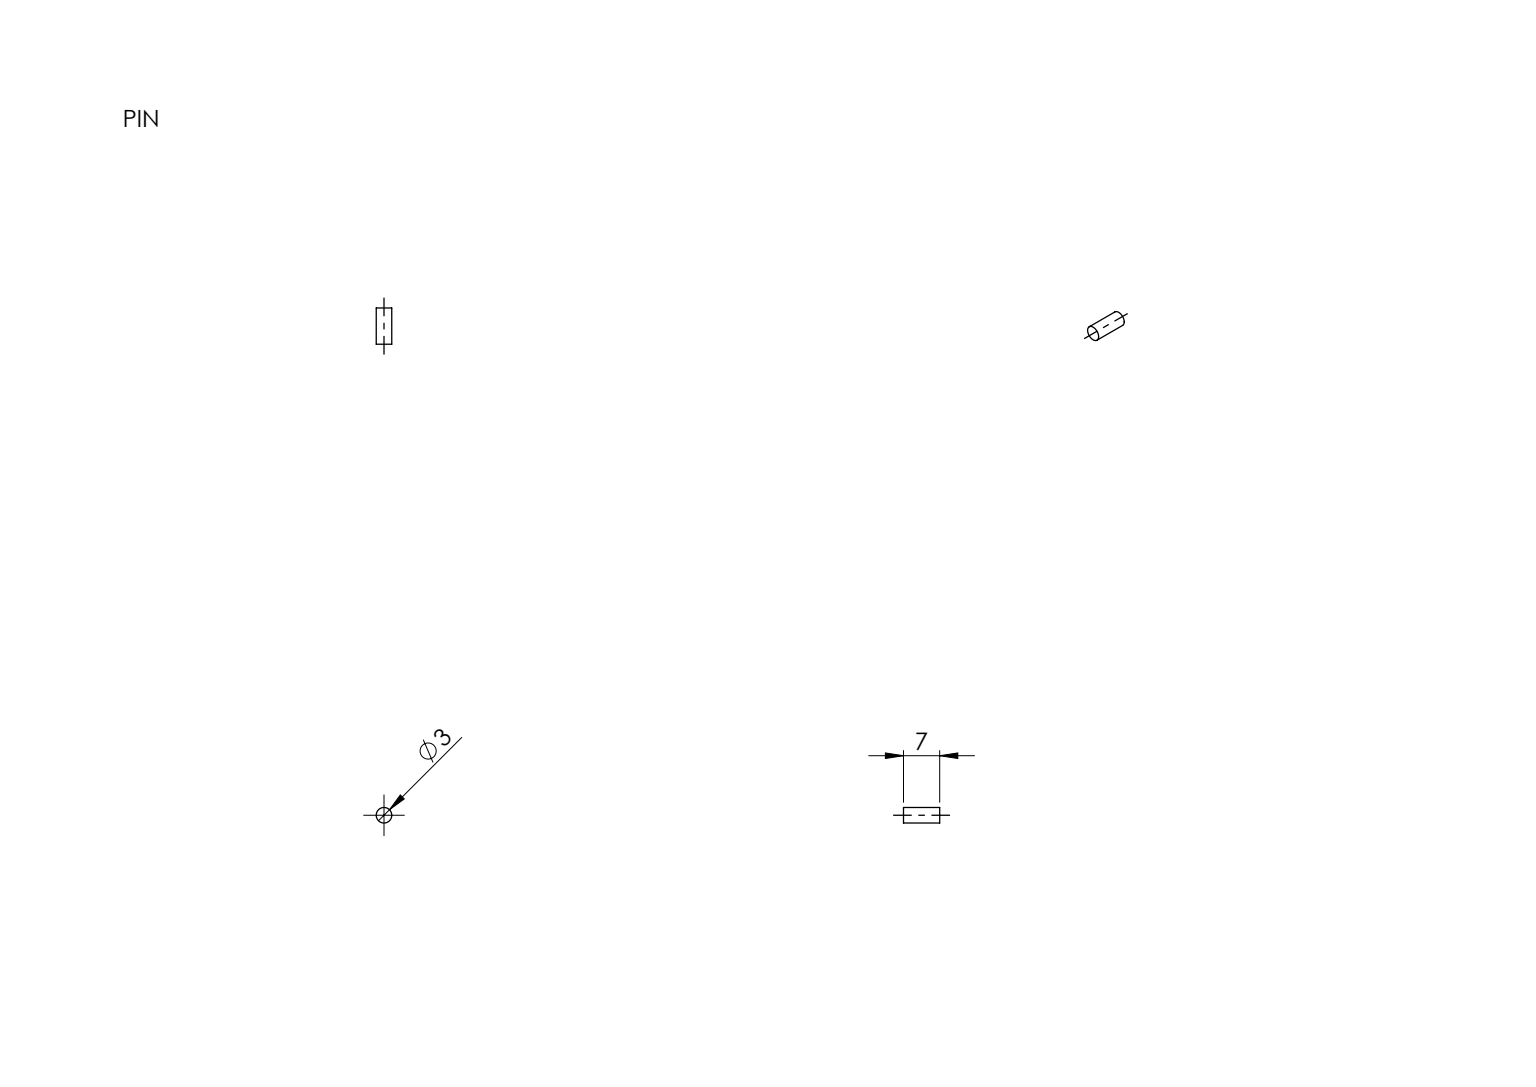
ISO-10303-21;
HEADER;
FILE_DESCRIPTION (('STEP AP214'),
    '1' );
FILE_NAME ('pin.step',
    '2026-10-04T07:56:41',
    ( '' ),
    ( '' ),
    'SwSTEP 2.0',
    'SolidWorks 2026',
    '' );
FILE_SCHEMA (( 'AUTOMOTIVE_DESIGN' ));
ENDSEC;

DATA;
#85=DIRECTION ( 'NONE',  ( 0.000000000000000000, 0.000000000000000000, 1.000000000000000000 ) ) ;
#302=UNCERTAINTY_MEASURE_WITH_UNIT (LENGTH_MEASURE( 1.000000000000000082E-05 ), #4684, 'distance_accuracy_value', 'NONE');
#316=ORIENTED_EDGE ( 'NONE', *, *, #6930, .F. ) ;
#319=AXIS2_PLACEMENT_3D ( 'NONE', #8320, #7056, #3853 ) ;
#388=( NAMED_UNIT ( * ) PLANE_ANGLE_UNIT ( ) SI_UNIT ( $, .RADIAN. ) );
#452=AXIS2_PLACEMENT_3D ( 'NONE', #3365, #5291, #5925 ) ;
#471=FILL_AREA_STYLE ('',( #4980 ) ) ;
#537=ORIENTED_EDGE ( 'NONE', *, *, #4750, .F. ) ;
#543=ADVANCED_FACE ( 'NONE', ( #3277 ), #2060, .T. ) ;
#563=PRODUCT_DEFINITION_SHAPE ( 'NONE', 'NONE',  #5357 ) ;
#690=CARTESIAN_POINT ( 'NONE',  ( -1.500000000000000666, -26.99999999999998934, -7.000000000000000000 ) ) ;
#723=FACE_OUTER_BOUND ( 'NONE', #8185, .T. ) ;
#897=SURFACE_STYLE_USAGE ( .BOTH. , #2921 ) ;
#985=SURFACE_STYLE_USAGE ( .BOTH. , #1105 ) ;
#1105=SURFACE_SIDE_STYLE ('',( #1786 ) ) ;
#1148=CLOSED_SHELL ( 'NONE', ( #543, #2137, #6595, #3524 ) ) ;
#1208=DIRECTION ( 'NONE',  ( 1.000000000000000000, 0.000000000000000000, -0.000000000000000000 ) ) ;
#1236=DIRECTION ( 'NONE',  ( 1.000000000000000000, 0.000000000000000000, 0.000000000000000000 ) ) ;
#1290=DIRECTION ( 'NONE',  ( 0.000000000000000000, 0.000000000000000000, 1.000000000000000000 ) ) ;
#1354=CARTESIAN_POINT ( 'NONE',  ( 6.123233995736760366E-16, -26.99999999999998934, 0.000000000000000000 ) ) ;
#1363=PLANE ( 'NONE',  #7305 ) ;
#1476=MECHANICAL_DESIGN_GEOMETRIC_PRESENTATION_REPRESENTATION('',(#7399),#3358);
#1613=SHAPE_REPRESENTATION ( 'pin', ( #2840 ), #2157 ) ;
#1657=( NAMED_UNIT ( * ) SI_UNIT ( $, .STERADIAN. ) SOLID_ANGLE_UNIT ( ) );
#1756=DIRECTION ( 'NONE',  ( 1.000000000000000000, 0.000000000000000000, 0.000000000000000000 ) ) ;
#1770=EDGE_LOOP ( 'NONE', ( #6300, #7373, #537, #2844 ) ) ;
#1786=SURFACE_STYLE_FILL_AREA ( #471 ) ;
#2029=EDGE_LOOP ( 'NONE', ( #4288, #7071 ) ) ;
#2060=CYLINDRICAL_SURFACE ( 'NONE', #452, 1.500000000000001332 ) ;
#2099=CARTESIAN_POINT ( 'NONE',  ( 1.500000000000001998, -26.99999999999998934, -7.000000000000000000 ) ) ;
#2137=ADVANCED_FACE ( 'NONE', ( #2897 ), #5462, .T. ) ;
#2157=( GEOMETRIC_REPRESENTATION_CONTEXT ( 3 ) GLOBAL_UNCERTAINTY_ASSIGNED_CONTEXT ( ( #302 ) ) GLOBAL_UNIT_ASSIGNED_CONTEXT ( ( #4684, #4862, #6834 ) ) REPRESENTATION_CONTEXT ( 'NONE', 'WORKASPACE' ) );
#2269=CARTESIAN_POINT ( 'NONE',  ( 6.123233995736760366E-16, -26.99999999999998934, -7.000000000000000000 ) ) ;
#2287=EDGE_CURVE ( 'NONE', #5238, #8124, #2354, .T. ) ;
#2354=CIRCLE ( 'NONE', #319, 1.500000000000001332 ) ;
#2380=( LENGTH_UNIT ( ) NAMED_UNIT ( * ) SI_UNIT ( .MILLI., .METRE. ) );
#2511=DIRECTION ( 'NONE',  ( 0.000000000000000000, 0.000000000000000000, 1.000000000000000000 ) ) ;
#2696=VECTOR ( 'NONE', #85, 1000.000000000000000 ) ;
#2840=AXIS2_PLACEMENT_3D ( 'NONE', #8120, #5497, #1756 ) ;
#2844=ORIENTED_EDGE ( 'NONE', *, *, #7496, .F. ) ;
#2879=COLOUR_RGB ( '', 0.72549020, 0.75294118, 0.79215686) ;
#2890=ADVANCED_BREP_SHAPE_REPRESENTATION ( '', ( #4458, #2840 ), #2157 ) ;
#2897=FACE_OUTER_BOUND ( 'NONE', #2937, .T. ) ;
#2921=SURFACE_SIDE_STYLE ('',( #7945 ) ) ;
#2935=ORIENTED_EDGE ( 'NONE', *, *, #2287, .T. ) ;
#2937=EDGE_LOOP ( 'NONE', ( #6441, #2935, #4800, #316 ) ) ;
#3085=CIRCLE ( 'NONE', #7803, 1.500000000000001332 ) ;
#3088=PRESENTATION_STYLE_ASSIGNMENT (( #985 ) ) ;
#3277=FACE_OUTER_BOUND ( 'NONE', #1770, .T. ) ;
#3300=CARTESIAN_POINT ( 'NONE',  ( 1.500000000000001998, -26.99999999999998934, -7.000000000000000000 ) ) ;
#3358=( GEOMETRIC_REPRESENTATION_CONTEXT ( 3 ) GLOBAL_UNCERTAINTY_ASSIGNED_CONTEXT ( ( #5447 ) ) GLOBAL_UNIT_ASSIGNED_CONTEXT ( ( #2380, #388, #3594 ) ) REPRESENTATION_CONTEXT ( 'NONE', 'WORKASPACE' ) );
#3365=CARTESIAN_POINT ( 'NONE',  ( 6.123233995736760366E-16, -26.99999999999998934, -7.000000000000000000 ) ) ;
#3379=EDGE_CURVE ( 'NONE', #8124, #5238, #8118, .T. ) ;
#3470=PRESENTATION_STYLE_ASSIGNMENT (( #897 ) ) ;
#3498=CARTESIAN_POINT ( 'NONE',  ( -1.500000000000000666, -26.99999999999998934, -7.000000000000000000 ) ) ;
#3524=ADVANCED_FACE ( 'NONE', ( #723 ), #1363, .T. ) ;
#3594=( NAMED_UNIT ( * ) SI_UNIT ( $, .STERADIAN. ) SOLID_ANGLE_UNIT ( ) );
#3818=CIRCLE ( 'NONE', #4761, 1.500000000000001332 ) ;
#3820=LINE ( 'NONE', #690, #4164 ) ;
#3853=DIRECTION ( 'NONE',  ( 1.000000000000000000, 0.000000000000000000, 0.000000000000000000 ) ) ;
#3939=PLANE ( 'NONE',  #5028 ) ;
#4026=COLOUR_RGB ( '', 0.72549020, 0.75294118, 0.79215686) ;
#4070=AXIS2_PLACEMENT_3D ( 'NONE', #4425, #7009, #1236 ) ;
#4092=MECHANICAL_DESIGN_GEOMETRIC_PRESENTATION_REPRESENTATION('',(#7728),#6103);
#4099=AXIS2_PLACEMENT_3D ( 'NONE', #2269, #7016, #4392 ) ;
#4164=VECTOR ( 'NONE', #1290, 1000.000000000000000 ) ;
#4288=ORIENTED_EDGE ( 'NONE', *, *, #3379, .F. ) ;
#4392=DIRECTION ( 'NONE',  ( 1.000000000000000000, 0.000000000000000000, 0.000000000000000000 ) ) ;
#4425=CARTESIAN_POINT ( 'NONE',  ( 6.123233995736760366E-16, -26.99999999999998934, -7.000000000000000000 ) ) ;
#4458=MANIFOLD_SOLID_BREP ( 'Boss-Extrude1', #1148 ) ;
#4479=CARTESIAN_POINT ( 'NONE',  ( -1.500000000000000666, -26.99999999999998934, 0.000000000000000000 ) ) ;
#4586=DIRECTION ( 'NONE',  ( 1.000000000000000000, 0.000000000000000000, 0.000000000000000000 ) ) ;
#4684=( LENGTH_UNIT ( ) NAMED_UNIT ( * ) SI_UNIT ( .MILLI., .METRE. ) );
#4750=EDGE_CURVE ( 'NONE', #5131, #6672, #3085, .T. ) ;
#4761=AXIS2_PLACEMENT_3D ( 'NONE', #4812, #7389, #5488 ) ;
#4768=PRODUCT_DEFINITION_CONTEXT ( 'detailed design', #6632, 'design' ) ;
#4769=FILL_AREA_STYLE ('',( #6159 ) ) ;
#4800=ORIENTED_EDGE ( 'NONE', *, *, #7496, .T. ) ;
#4812=CARTESIAN_POINT ( 'NONE',  ( 6.123233995736760366E-16, -26.99999999999998934, 0.000000000000000000 ) ) ;
#4862=( NAMED_UNIT ( * ) PLANE_ANGLE_UNIT ( ) SI_UNIT ( $, .RADIAN. ) );
#4899=( LENGTH_UNIT ( ) NAMED_UNIT ( * ) SI_UNIT ( .MILLI., .METRE. ) );
#4905=SHAPE_REPRESENTATION_RELATIONSHIP ( 'NONE' , 'NONE' ,  #1613, #2890 ) ;
#4980=FILL_AREA_STYLE_COLOUR ( '', #4026 ) ;
#5028=AXIS2_PLACEMENT_3D ( 'NONE', #6973, #2511, #1208 ) ;
#5131=VERTEX_POINT ( 'NONE', #7975 ) ;
#5238=VERTEX_POINT ( 'NONE', #3498 ) ;
#5291=DIRECTION ( 'NONE',  ( 0.000000000000000000, 0.000000000000000000, 1.000000000000000000 ) ) ;
#5357=PRODUCT_DEFINITION ( 'UNKNOWN', '', #7127, #4768 ) ;
#5447=UNCERTAINTY_MEASURE_WITH_UNIT (LENGTH_MEASURE( 1.000000000000000082E-05 ), #2380, 'distance_accuracy_value', 'NONE');
#5462=CYLINDRICAL_SURFACE ( 'NONE', #4099, 1.500000000000001332 ) ;
#5488=DIRECTION ( 'NONE',  ( 1.000000000000000000, 0.000000000000000000, 0.000000000000000000 ) ) ;
#5497=DIRECTION ( 'NONE',  ( 0.000000000000000000, 0.000000000000000000, 1.000000000000000000 ) ) ;
#5766=APPLICATION_CONTEXT ( 'automotive_design' ) ;
#5863=DIRECTION ( 'NONE',  ( 0.000000000000000000, 0.000000000000000000, 1.000000000000000000 ) ) ;
#5925=DIRECTION ( 'NONE',  ( 1.000000000000000000, 0.000000000000000000, 0.000000000000000000 ) ) ;
#6037=( NAMED_UNIT ( * ) PLANE_ANGLE_UNIT ( ) SI_UNIT ( $, .RADIAN. ) );
#6103=( GEOMETRIC_REPRESENTATION_CONTEXT ( 3 ) GLOBAL_UNCERTAINTY_ASSIGNED_CONTEXT ( ( #7487 ) ) GLOBAL_UNIT_ASSIGNED_CONTEXT ( ( #4899, #6037, #1657 ) ) REPRESENTATION_CONTEXT ( 'NONE', 'WORKASPACE' ) );
#6159=FILL_AREA_STYLE_COLOUR ( '', #2879 ) ;
#6217=PRODUCT ( 'pin', 'pin', '', ( #8280 ) ) ;
#6300=ORIENTED_EDGE ( 'NONE', *, *, #3379, .T. ) ;
#6348=FACE_OUTER_BOUND ( 'NONE', #2029, .T. ) ;
#6441=ORIENTED_EDGE ( 'NONE', *, *, #8026, .F. ) ;
#6451=DIRECTION ( 'NONE',  ( 0.000000000000000000, 0.000000000000000000, 1.000000000000000000 ) ) ;
#6480=ORIENTED_EDGE ( 'NONE', *, *, #6930, .T. ) ;
#6595=ADVANCED_FACE ( 'NONE', ( #6348 ), #3939, .F. ) ;
#6632=APPLICATION_CONTEXT ( 'automotive_design' ) ;
#6672=VERTEX_POINT ( 'NONE', #4479 ) ;
#6834=( NAMED_UNIT ( * ) SI_UNIT ( $, .STERADIAN. ) SOLID_ANGLE_UNIT ( ) );
#6930=EDGE_CURVE ( 'NONE', #6672, #5131, #3818, .T. ) ;
#6971=SHAPE_DEFINITION_REPRESENTATION ( #563, #1613 ) ;
#6973=CARTESIAN_POINT ( 'NONE',  ( 6.123233995736760366E-16, -26.99999999999998934, -7.000000000000000000 ) ) ;
#7009=DIRECTION ( 'NONE',  ( 0.000000000000000000, 0.000000000000000000, 1.000000000000000000 ) ) ;
#7016=DIRECTION ( 'NONE',  ( 0.000000000000000000, 0.000000000000000000, 1.000000000000000000 ) ) ;
#7056=DIRECTION ( 'NONE',  ( 0.000000000000000000, 0.000000000000000000, 1.000000000000000000 ) ) ;
#7071=ORIENTED_EDGE ( 'NONE', *, *, #2287, .F. ) ;
#7127=PRODUCT_DEFINITION_FORMATION_WITH_SPECIFIED_SOURCE ( 'ANY', '', #6217, .NOT_KNOWN. ) ;
#7137=CARTESIAN_POINT ( 'NONE',  ( 6.123233995736760366E-16, -26.99999999999998934, 0.000000000000000000 ) ) ;
#7215=LINE ( 'NONE', #3300, #2696 ) ;
#7305=AXIS2_PLACEMENT_3D ( 'NONE', #7137, #5863, #7815 ) ;
#7373=ORIENTED_EDGE ( 'NONE', *, *, #8026, .T. ) ;
#7389=DIRECTION ( 'NONE',  ( 0.000000000000000000, 0.000000000000000000, 1.000000000000000000 ) ) ;
#7399=STYLED_ITEM ( 'NONE', ( #3088 ), #2890 ) ;
#7487=UNCERTAINTY_MEASURE_WITH_UNIT (LENGTH_MEASURE( 1.000000000000000082E-05 ), #4899, 'distance_accuracy_value', 'NONE');
#7496=EDGE_CURVE ( 'NONE', #8124, #5131, #7215, .T. ) ;
#7728=STYLED_ITEM ( 'NONE', ( #3470 ), #4458 ) ;
#7803=AXIS2_PLACEMENT_3D ( 'NONE', #1354, #6451, #4586 ) ;
#7815=DIRECTION ( 'NONE',  ( 1.000000000000000000, 0.000000000000000000, -0.000000000000000000 ) ) ;
#7842=ORIENTED_EDGE ( 'NONE', *, *, #4750, .T. ) ;
#7945=SURFACE_STYLE_FILL_AREA ( #4769 ) ;
#7975=CARTESIAN_POINT ( 'NONE',  ( 1.500000000000001998, -26.99999999999998934, 0.000000000000000000 ) ) ;
#8026=EDGE_CURVE ( 'NONE', #5238, #6672, #3820, .T. ) ;
#8118=CIRCLE ( 'NONE', #4070, 1.500000000000001332 ) ;
#8120=CARTESIAN_POINT ( 'NONE',  ( 0.000000000000000000, 0.000000000000000000, 0.000000000000000000 ) ) ;
#8124=VERTEX_POINT ( 'NONE', #2099 ) ;
#8185=EDGE_LOOP ( 'NONE', ( #7842, #6480 ) ) ;
#8280=PRODUCT_CONTEXT ( 'NONE', #5766, 'mechanical' ) ;
#8320=CARTESIAN_POINT ( 'NONE',  ( 6.123233995736760366E-16, -26.99999999999998934, -7.000000000000000000 ) ) ;
ENDSEC;
END-ISO-10303-21;
